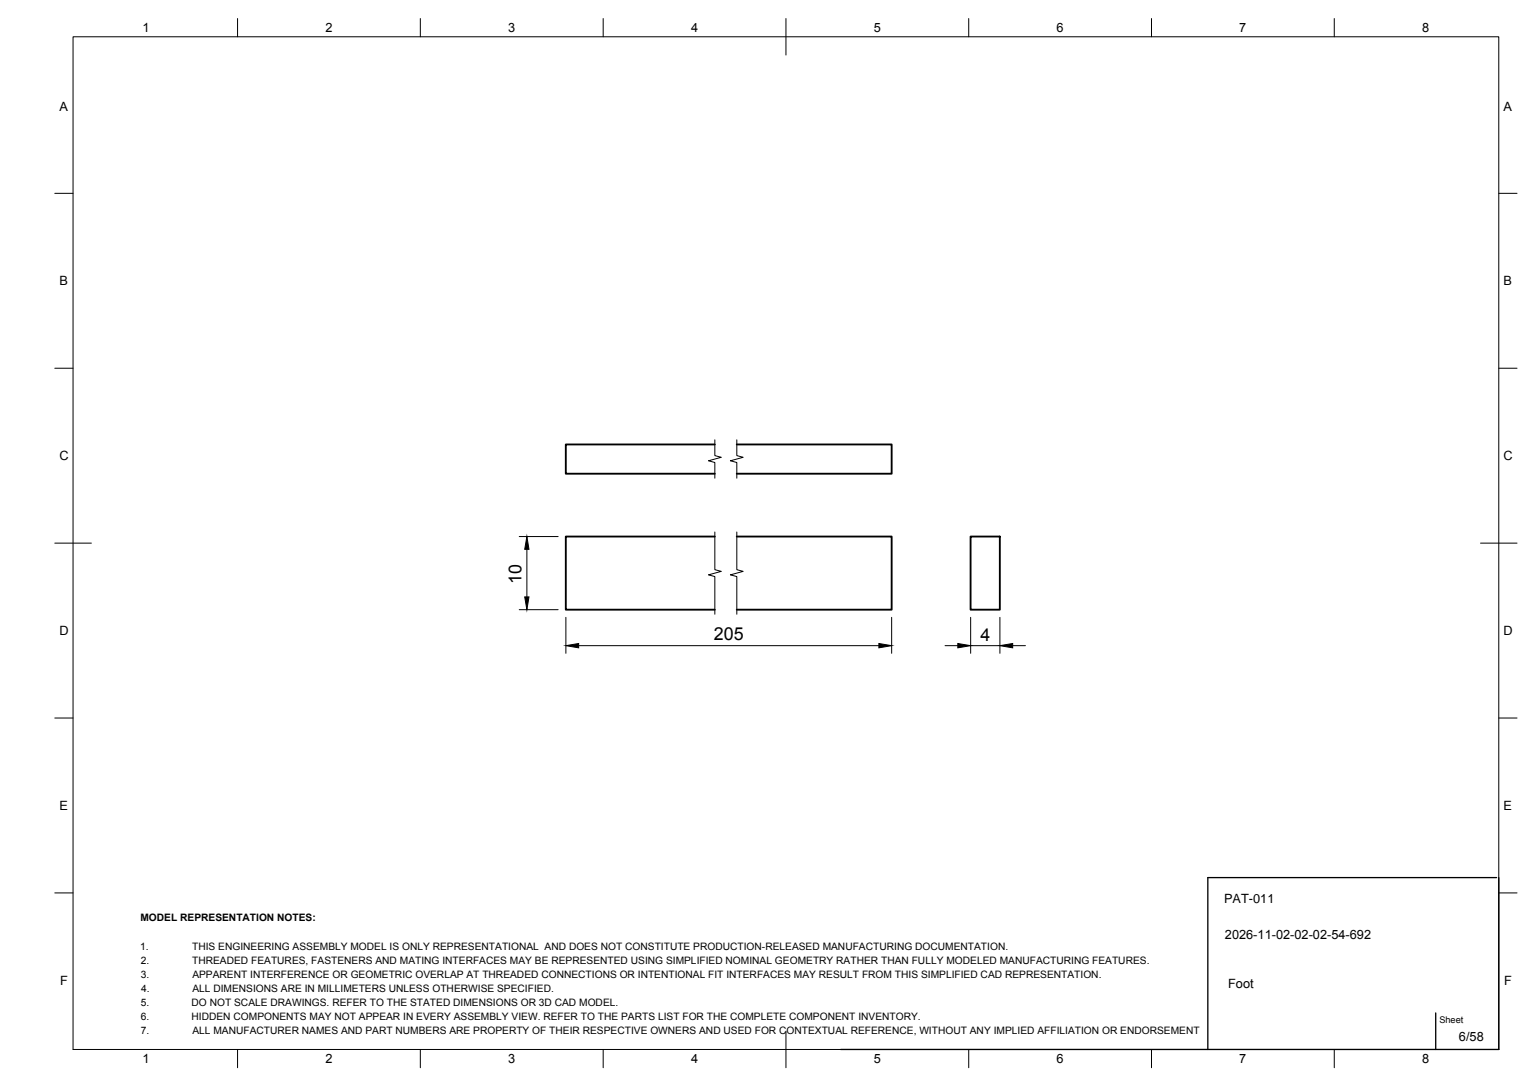
ISO-10303-21;
HEADER;
/* Generated by software containing ST-Developer
 * from STEP Tools, Inc. (www.steptools.com) 
 */

FILE_DESCRIPTION(
/* description */ ('Belt tension measurement rig'),
/* implementation_level */ '2;1');

FILE_NAME(
/* name */ 'Foot.step',
/* time_stamp */ '2026-10-28T03:24:44-07:00',
/* author */ (''),
/* organization */ (''),
/* preprocessor_version */ 'ST-DEVELOPER v20.2',
/* originating_system */ 'Autodesk Translation Framework v15.17.0.0',
/* authorisation */ '');

FILE_SCHEMA (('AUTOMOTIVE_DESIGN { 1 0 10303 214 3 1 1 }'));
ENDSEC;

DATA;
#10=MECHANICAL_DESIGN_GEOMETRIC_PRESENTATION_REPRESENTATION('',(#693),#23587);
#583=SHAPE_REPRESENTATION_RELATIONSHIP('SRR','None',#23828,#638);
#638=ADVANCED_BREP_SHAPE_REPRESENTATION('',(#763),#23526);
#693=STYLED_ITEM('',(#24225),#763);
#763=MANIFOLD_SOLID_BREP('Body1',#12198);
#1057=PLANE('',#12942);
#1058=PLANE('',#12943);
#1059=PLANE('',#12944);
#1060=PLANE('',#12945);
#1061=PLANE('',#12946);
#1062=PLANE('',#12947);
#1386=FACE_OUTER_BOUND('',#2104,.T.);
#1387=FACE_OUTER_BOUND('',#2105,.T.);
#1388=FACE_OUTER_BOUND('',#2106,.T.);
#1389=FACE_OUTER_BOUND('',#2107,.T.);
#1390=FACE_OUTER_BOUND('',#2108,.T.);
#1391=FACE_OUTER_BOUND('',#2109,.T.);
#2104=EDGE_LOOP('',(#8046,#8047,#8048,#8049));
#2105=EDGE_LOOP('',(#8050,#8051,#8052,#8053));
#2106=EDGE_LOOP('',(#8054,#8055,#8056,#8057));
#2107=EDGE_LOOP('',(#8058,#8059,#8060,#8061));
#2108=EDGE_LOOP('',(#8062,#8063,#8064,#8065));
#2109=EDGE_LOOP('',(#8066,#8067,#8068,#8069));
#2994=LINE('',#18681,#3745);
#2995=LINE('',#18683,#3746);
#2996=LINE('',#18685,#3747);
#2997=LINE('',#18686,#3748);
#2998=LINE('',#18689,#3749);
#2999=LINE('',#18691,#3750);
#3000=LINE('',#18692,#3751);
#3001=LINE('',#18695,#3752);
#3002=LINE('',#18697,#3753);
#3003=LINE('',#18698,#3754);
#3004=LINE('',#18700,#3755);
#3005=LINE('',#18701,#3756);
#3745=VECTOR('',#14677,1.);
#3746=VECTOR('',#14678,1.);
#3747=VECTOR('',#14679,1.);
#3748=VECTOR('',#14680,1.);
#3749=VECTOR('',#14683,1.);
#3750=VECTOR('',#14684,1.);
#3751=VECTOR('',#14685,1.);
#3752=VECTOR('',#14688,1.);
#3753=VECTOR('',#14689,1.);
#3754=VECTOR('',#14690,1.);
#3755=VECTOR('',#14693,1.);
#3756=VECTOR('',#14694,1.);
#5274=VERTEX_POINT('',#18679);
#5275=VERTEX_POINT('',#18680);
#5276=VERTEX_POINT('',#18682);
#5277=VERTEX_POINT('',#18684);
#5278=VERTEX_POINT('',#18688);
#5279=VERTEX_POINT('',#18690);
#5280=VERTEX_POINT('',#18694);
#5281=VERTEX_POINT('',#18696);
#6382=EDGE_CURVE('',#5274,#5275,#2994,.T.);
#6383=EDGE_CURVE('',#5275,#5276,#2995,.T.);
#6384=EDGE_CURVE('',#5277,#5276,#2996,.T.);
#6385=EDGE_CURVE('',#5274,#5277,#2997,.T.);
#6386=EDGE_CURVE('',#5278,#5274,#2998,.T.);
#6387=EDGE_CURVE('',#5279,#5277,#2999,.T.);
#6388=EDGE_CURVE('',#5278,#5279,#3000,.T.);
#6389=EDGE_CURVE('',#5280,#5278,#3001,.T.);
#6390=EDGE_CURVE('',#5281,#5279,#3002,.T.);
#6391=EDGE_CURVE('',#5280,#5281,#3003,.T.);
#6392=EDGE_CURVE('',#5275,#5280,#3004,.T.);
#6393=EDGE_CURVE('',#5276,#5281,#3005,.T.);
#8046=ORIENTED_EDGE('',*,*,#6382,.T.);
#8047=ORIENTED_EDGE('',*,*,#6383,.T.);
#8048=ORIENTED_EDGE('',*,*,#6384,.F.);
#8049=ORIENTED_EDGE('',*,*,#6385,.F.);
#8050=ORIENTED_EDGE('',*,*,#6386,.T.);
#8051=ORIENTED_EDGE('',*,*,#6385,.T.);
#8052=ORIENTED_EDGE('',*,*,#6387,.F.);
#8053=ORIENTED_EDGE('',*,*,#6388,.F.);
#8054=ORIENTED_EDGE('',*,*,#6389,.T.);
#8055=ORIENTED_EDGE('',*,*,#6388,.T.);
#8056=ORIENTED_EDGE('',*,*,#6390,.F.);
#8057=ORIENTED_EDGE('',*,*,#6391,.F.);
#8058=ORIENTED_EDGE('',*,*,#6392,.T.);
#8059=ORIENTED_EDGE('',*,*,#6391,.T.);
#8060=ORIENTED_EDGE('',*,*,#6393,.F.);
#8061=ORIENTED_EDGE('',*,*,#6383,.F.);
#8062=ORIENTED_EDGE('',*,*,#6393,.T.);
#8063=ORIENTED_EDGE('',*,*,#6390,.T.);
#8064=ORIENTED_EDGE('',*,*,#6387,.T.);
#8065=ORIENTED_EDGE('',*,*,#6384,.T.);
#8066=ORIENTED_EDGE('',*,*,#6392,.F.);
#8067=ORIENTED_EDGE('',*,*,#6382,.F.);
#8068=ORIENTED_EDGE('',*,*,#6386,.F.);
#8069=ORIENTED_EDGE('',*,*,#6389,.F.);
#11527=ADVANCED_FACE('',(#1386),#1057,.T.);
#11528=ADVANCED_FACE('',(#1387),#1058,.T.);
#11529=ADVANCED_FACE('',(#1388),#1059,.T.);
#11530=ADVANCED_FACE('',(#1389),#1060,.T.);
#11531=ADVANCED_FACE('',(#1390),#1061,.T.);
#11532=ADVANCED_FACE('',(#1391),#1062,.F.);
#12198=CLOSED_SHELL('',(#11527,#11528,#11529,#11530,#11531,#11532));
#12941=AXIS2_PLACEMENT_3D('',#18677,#14673,#14674);
#12942=AXIS2_PLACEMENT_3D('',#18678,#14675,#14676);
#12943=AXIS2_PLACEMENT_3D('',#18687,#14681,#14682);
#12944=AXIS2_PLACEMENT_3D('',#18693,#14686,#14687);
#12945=AXIS2_PLACEMENT_3D('',#18699,#14691,#14692);
#12946=AXIS2_PLACEMENT_3D('',#18702,#14695,#14696);
#12947=AXIS2_PLACEMENT_3D('',#18703,#14697,#14698);
#14673=DIRECTION('axis',(0.,0.,1.));
#14674=DIRECTION('refdir',(1.,0.,0.));
#14675=DIRECTION('center_axis',(0.,1.,0.));
#14676=DIRECTION('ref_axis',(-1.,0.,0.));
#14677=DIRECTION('',(-1.,0.,0.));
#14678=DIRECTION('',(0.,0.,1.));
#14679=DIRECTION('',(-1.,0.,0.));
#14680=DIRECTION('',(0.,0.,1.));
#14681=DIRECTION('center_axis',(1.,0.,0.));
#14682=DIRECTION('ref_axis',(0.,1.,0.));
#14683=DIRECTION('',(0.,1.,0.));
#14684=DIRECTION('',(0.,1.,0.));
#14685=DIRECTION('',(0.,0.,1.));
#14686=DIRECTION('center_axis',(0.,-1.,0.));
#14687=DIRECTION('ref_axis',(1.,0.,0.));
#14688=DIRECTION('',(1.,0.,0.));
#14689=DIRECTION('',(1.,0.,0.));
#14690=DIRECTION('',(0.,0.,1.));
#14691=DIRECTION('center_axis',(-1.,0.,0.));
#14692=DIRECTION('ref_axis',(0.,-1.,0.));
#14693=DIRECTION('',(0.,-1.,0.));
#14694=DIRECTION('',(0.,-1.,0.));
#14695=DIRECTION('center_axis',(0.,0.,1.));
#14696=DIRECTION('ref_axis',(1.,0.,0.));
#14697=DIRECTION('center_axis',(0.,0.,1.));
#14698=DIRECTION('ref_axis',(1.,0.,0.));
#18677=CARTESIAN_POINT('',(0.,0.,0.));
#18678=CARTESIAN_POINT('Origin',(-1.5,14.,-1.6));
#18679=CARTESIAN_POINT('',(-1.5,14.,-1.6));
#18680=CARTESIAN_POINT('',(-2.5,14.,-1.6));
#18681=CARTESIAN_POINT('',(-1.5,14.,-1.6));
#18682=CARTESIAN_POINT('',(-2.5,14.,-1.2));
#18683=CARTESIAN_POINT('',(-2.5,14.,-1.6));
#18684=CARTESIAN_POINT('',(-1.5,14.,-1.2));
#18685=CARTESIAN_POINT('',(-1.5,14.,-1.2));
#18686=CARTESIAN_POINT('',(-1.5,14.,-1.6));
#18687=CARTESIAN_POINT('Origin',(-1.5,-6.5,-1.6));
#18688=CARTESIAN_POINT('',(-1.5,-6.5,-1.6));
#18689=CARTESIAN_POINT('',(-1.5,-6.5,-1.6));
#18690=CARTESIAN_POINT('',(-1.5,-6.5,-1.2));
#18691=CARTESIAN_POINT('',(-1.5,-6.5,-1.2));
#18692=CARTESIAN_POINT('',(-1.5,-6.5,-1.6));
#18693=CARTESIAN_POINT('Origin',(-2.5,-6.5,-1.6));
#18694=CARTESIAN_POINT('',(-2.5,-6.5,-1.6));
#18695=CARTESIAN_POINT('',(-2.5,-6.5,-1.6));
#18696=CARTESIAN_POINT('',(-2.5,-6.5,-1.2));
#18697=CARTESIAN_POINT('',(-2.5,-6.5,-1.2));
#18698=CARTESIAN_POINT('',(-2.5,-6.5,-1.6));
#18699=CARTESIAN_POINT('Origin',(-2.5,14.,-1.6));
#18700=CARTESIAN_POINT('',(-2.5,14.,-1.6));
#18701=CARTESIAN_POINT('',(-2.5,14.,-1.2));
#18702=CARTESIAN_POINT('Origin',(-2.,3.75,-1.2));
#18703=CARTESIAN_POINT('Origin',(-2.,3.75,-1.6));
#23461=UNCERTAINTY_MEASURE_WITH_UNIT(LENGTH_MEASURE(0.001),#23588,
'DISTANCE_ACCURACY_VALUE',
'Maximum model space distance between geometric entities at asserted c
onnectivities');
#23522=UNCERTAINTY_MEASURE_WITH_UNIT(LENGTH_MEASURE(0.001),#23588,
'DISTANCE_ACCURACY_VALUE',
'Maximum model space distance between geometric entities at asserted c
onnectivities');
#23526=(
GEOMETRIC_REPRESENTATION_CONTEXT(3)
GLOBAL_UNCERTAINTY_ASSIGNED_CONTEXT((#23461))
GLOBAL_UNIT_ASSIGNED_CONTEXT((#23588,#23590,#23591))
REPRESENTATION_CONTEXT('','3D')
);
#23587=(
GEOMETRIC_REPRESENTATION_CONTEXT(3)
GLOBAL_UNCERTAINTY_ASSIGNED_CONTEXT((#23522))
GLOBAL_UNIT_ASSIGNED_CONTEXT((#23588,#23590,#23591))
REPRESENTATION_CONTEXT('','3D')
);
#23588=(
LENGTH_UNIT()
NAMED_UNIT(*)
SI_UNIT(.CENTI.,.METRE.)
);
#23590=(
NAMED_UNIT(*)
PLANE_ANGLE_UNIT()
SI_UNIT($,.RADIAN.)
);
#23591=(
NAMED_UNIT(*)
SI_UNIT($,.STERADIAN.)
SOLID_ANGLE_UNIT()
);
#23595=SHAPE_DEFINITION_REPRESENTATION(#23659,#23828);
#23659=PRODUCT_DEFINITION_SHAPE('',$,#23893);
#23828=SHAPE_REPRESENTATION('',(#12941),#23526);
#23889=PRODUCT_DEFINITION_CONTEXT('part definition',#24083,'design');
#23893=PRODUCT_DEFINITION('Foot','Foot',#23957,#23889);
#23957=PRODUCT_DEFINITION_FORMATION('',$,#24088);
#24083=APPLICATION_CONTEXT(
'Core Data for Automotive Mechanical Design Process');
#24084=PRODUCT_CONTEXT('part definition',#24083,'mechanical');
#24088=PRODUCT('Foot','Foot','Foot',(#24084));
#24219=COLOUR_RGB('Off White',0.89,0.88,0.83);
#24220=FILL_AREA_STYLE_COLOUR('',#24219);
#24221=FILL_AREA_STYLE('',(#24220));
#24222=SURFACE_STYLE_FILL_AREA(#24221);
#24223=SURFACE_SIDE_STYLE('',(#24222));
#24224=SURFACE_STYLE_USAGE(.BOTH.,#24223);
#24225=PRESENTATION_STYLE_ASSIGNMENT((#24224));
ENDSEC;
END-ISO-10303-21;
